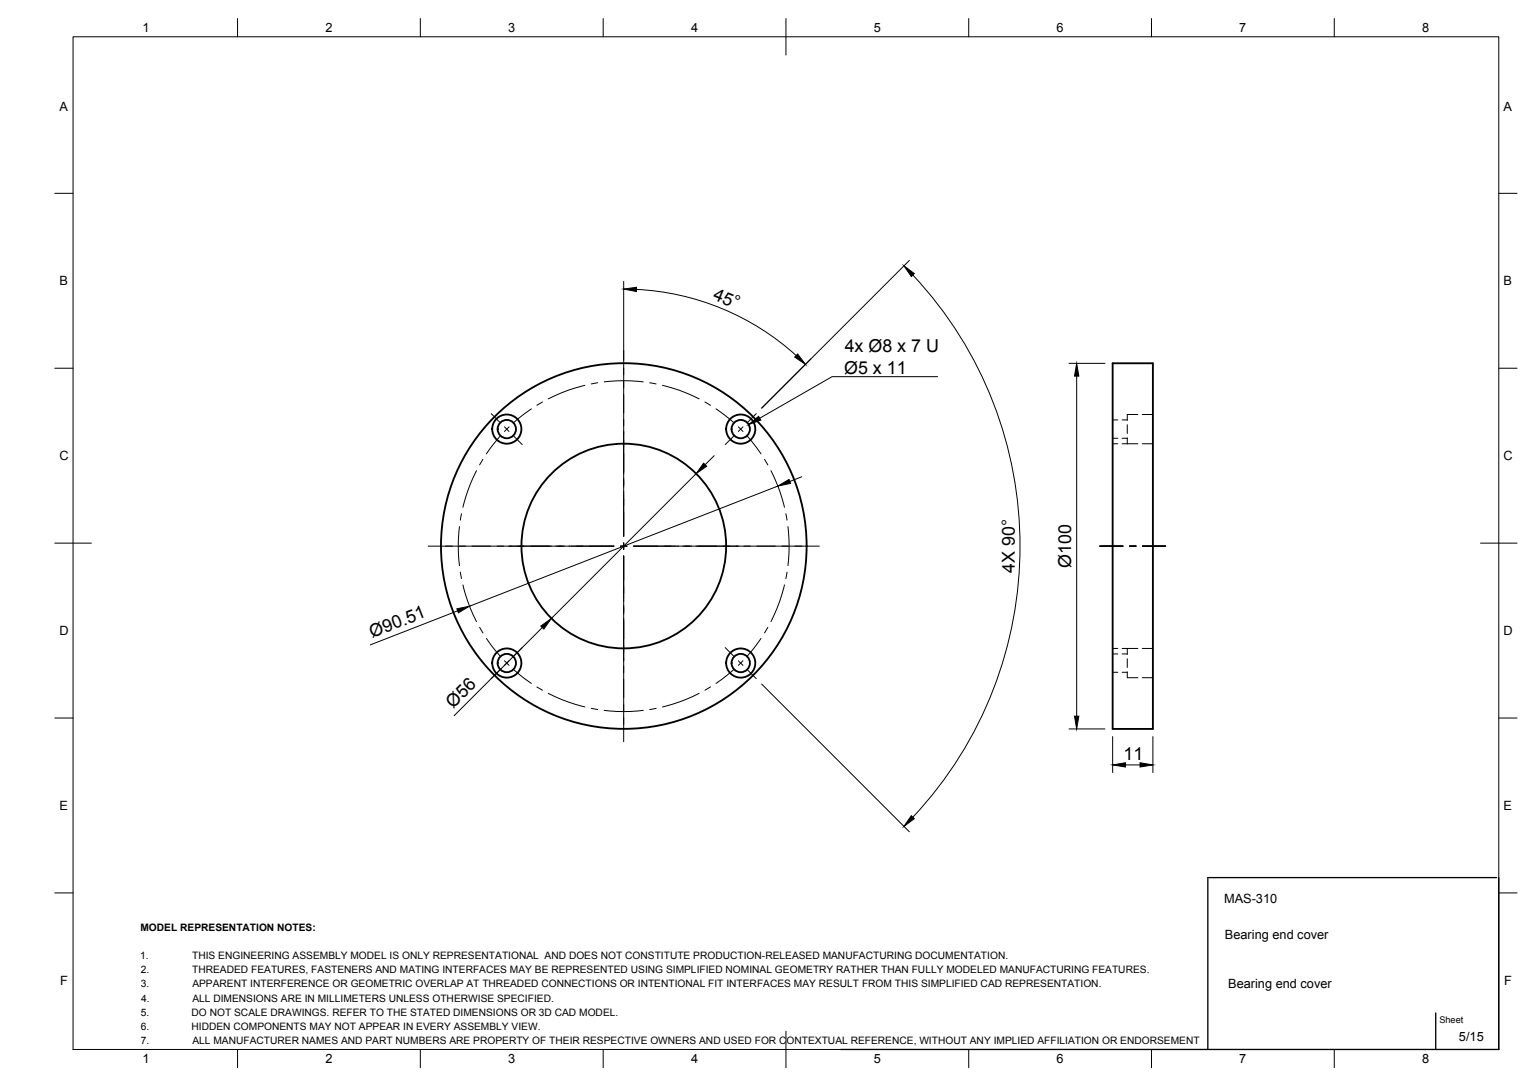
ISO-10303-21;
HEADER;
/* Generated by software containing ST-Developer
 * from STEP Tools, Inc. (www.steptools.com) 
 */

FILE_DESCRIPTION(
/* description */ ('Independent30mm screw-fed quill/spindle unit with16mm straight tool s
ocket, radial set screw, native reusable open ball bearings, retained 
inner/outer race stacks, keyed quill guide and M12x1.75 fine feed. Ext
ernal moving drive and tool not included. Ideal cage orbital links; in
dividual ball spin, force and preload not simulated. No drilling capac
ity, runout, speed, torque, load, life or machine safety rating.'),
/* implementation_level */ '2;1');

FILE_NAME(
/* name */ 'Bearing end cover.step',
/* time_stamp */ '2026-11-08T18:59:42-08:00',
/* author */ (''),
/* organization */ (''),
/* preprocessor_version */ 'ST-DEVELOPER v20.2',
/* originating_system */ 'Autodesk Translation Framework v15.17.0.0',
/* authorisation */ '');

FILE_SCHEMA (('AUTOMOTIVE_DESIGN { 1 0 10303 214 3 1 1 }'));
ENDSEC;

DATA;
#10=MECHANICAL_DESIGN_GEOMETRIC_PRESENTATION_REPRESENTATION('',(#1603),#63898);
#1567=SHAPE_REPRESENTATION_RELATIONSHIP('SRR','None',#64006,#1585);
#1585=ADVANCED_BREP_SHAPE_REPRESENTATION('',(#1621),#63891);
#1603=STYLED_ITEM('',(#64101),#1621);
#1621=MANIFOLD_SOLID_BREP('Body1',#15489);
#1692=FACE_BOUND('',#4293,.T.);
#1693=FACE_BOUND('',#4297,.T.);
#1694=FACE_BOUND('',#4301,.T.);
#1695=FACE_BOUND('',#4305,.T.);
#1696=FACE_BOUND('',#4311,.T.);
#1697=FACE_BOUND('',#4312,.T.);
#1698=FACE_BOUND('',#4313,.T.);
#1699=FACE_BOUND('',#4314,.T.);
#1700=FACE_BOUND('',#4315,.T.);
#1701=FACE_BOUND('',#4317,.T.);
#1702=FACE_BOUND('',#4318,.T.);
#1703=FACE_BOUND('',#4319,.T.);
#1704=FACE_BOUND('',#4320,.T.);
#1705=FACE_BOUND('',#4321,.T.);
#2325=CYLINDRICAL_SURFACE('',#16587,4.);
#2326=CYLINDRICAL_SURFACE('',#16589,2.5);
#2327=CYLINDRICAL_SURFACE('',#16594,4.);
#2328=CYLINDRICAL_SURFACE('',#16596,2.5);
#2329=CYLINDRICAL_SURFACE('',#16601,4.);
#2330=CYLINDRICAL_SURFACE('',#16603,2.5);
#2331=CYLINDRICAL_SURFACE('',#16608,4.);
#2332=CYLINDRICAL_SURFACE('',#16610,2.5);
#2333=CYLINDRICAL_SURFACE('',#16612,28.);
#2334=CYLINDRICAL_SURFACE('',#16615,50.);
#2550=CIRCLE('',#16585,4.);
#2551=CIRCLE('',#16586,2.5);
#2552=CIRCLE('',#16588,4.);
#2553=CIRCLE('',#16590,2.5);
#2554=CIRCLE('',#16592,4.);
#2555=CIRCLE('',#16593,2.5);
#2556=CIRCLE('',#16595,4.);
#2557=CIRCLE('',#16597,2.5);
#2558=CIRCLE('',#16599,4.);
#2559=CIRCLE('',#16600,2.5);
#2560=CIRCLE('',#16602,4.);
#2561=CIRCLE('',#16604,2.5);
#2562=CIRCLE('',#16606,4.);
#2563=CIRCLE('',#16607,2.5);
#2564=CIRCLE('',#16609,4.);
#2565=CIRCLE('',#16611,2.5);
#2566=CIRCLE('',#16613,28.);
#2567=CIRCLE('',#16614,28.);
#2568=CIRCLE('',#16616,50.);
#2569=CIRCLE('',#16617,50.);
#3390=FACE_OUTER_BOUND('',#4292,.T.);
#3391=FACE_OUTER_BOUND('',#4294,.T.);
#3392=FACE_OUTER_BOUND('',#4295,.T.);
#3393=FACE_OUTER_BOUND('',#4296,.T.);
#3394=FACE_OUTER_BOUND('',#4298,.T.);
#3395=FACE_OUTER_BOUND('',#4299,.T.);
#3396=FACE_OUTER_BOUND('',#4300,.T.);
#3397=FACE_OUTER_BOUND('',#4302,.T.);
#3398=FACE_OUTER_BOUND('',#4303,.T.);
#3399=FACE_OUTER_BOUND('',#4304,.T.);
#3400=FACE_OUTER_BOUND('',#4306,.T.);
#3401=FACE_OUTER_BOUND('',#4307,.T.);
#3402=FACE_OUTER_BOUND('',#4308,.T.);
#3403=FACE_OUTER_BOUND('',#4309,.T.);
#3404=FACE_OUTER_BOUND('',#4310,.T.);
#3405=FACE_OUTER_BOUND('',#4316,.T.);
#4292=EDGE_LOOP('',(#13930));
#4293=EDGE_LOOP('',(#13931));
#4294=EDGE_LOOP('',(#13932,#13933,#13934,#13935));
#4295=EDGE_LOOP('',(#13936,#13937,#13938,#13939));
#4296=EDGE_LOOP('',(#13940));
#4297=EDGE_LOOP('',(#13941));
#4298=EDGE_LOOP('',(#13942,#13943,#13944,#13945));
#4299=EDGE_LOOP('',(#13946,#13947,#13948,#13949));
#4300=EDGE_LOOP('',(#13950));
#4301=EDGE_LOOP('',(#13951));
#4302=EDGE_LOOP('',(#13952,#13953,#13954,#13955));
#4303=EDGE_LOOP('',(#13956,#13957,#13958,#13959));
#4304=EDGE_LOOP('',(#13960));
#4305=EDGE_LOOP('',(#13961));
#4306=EDGE_LOOP('',(#13962,#13963,#13964,#13965));
#4307=EDGE_LOOP('',(#13966,#13967,#13968,#13969));
#4308=EDGE_LOOP('',(#13970,#13971,#13972,#13973));
#4309=EDGE_LOOP('',(#13974,#13975,#13976,#13977));
#4310=EDGE_LOOP('',(#13978));
#4311=EDGE_LOOP('',(#13979));
#4312=EDGE_LOOP('',(#13980));
#4313=EDGE_LOOP('',(#13981));
#4314=EDGE_LOOP('',(#13982));
#4315=EDGE_LOOP('',(#13983));
#4316=EDGE_LOOP('',(#13984));
#4317=EDGE_LOOP('',(#13985));
#4318=EDGE_LOOP('',(#13986));
#4319=EDGE_LOOP('',(#13987));
#4320=EDGE_LOOP('',(#13988));
#4321=EDGE_LOOP('',(#13989));
#5114=LINE('',#60321,#5877);
#5115=LINE('',#60324,#5878);
#5116=LINE('',#60334,#5879);
#5117=LINE('',#60337,#5880);
#5118=LINE('',#60347,#5881);
#5119=LINE('',#60350,#5882);
#5120=LINE('',#60360,#5883);
#5121=LINE('',#60363,#5884);
#5122=LINE('',#60369,#5885);
#5123=LINE('',#60375,#5886);
#5877=VECTOR('',#19338,4.);
#5878=VECTOR('',#19341,2.5);
#5879=VECTOR('',#19354,4.);
#5880=VECTOR('',#19357,2.5);
#5881=VECTOR('',#19370,4.);
#5882=VECTOR('',#19373,2.5);
#5883=VECTOR('',#19386,4.);
#5884=VECTOR('',#19389,2.5);
#5885=VECTOR('',#19396,28.);
#5886=VECTOR('',#19403,50.);
#7310=VERTEX_POINT('',#60314);
#7311=VERTEX_POINT('',#60316);
#7312=VERTEX_POINT('',#60319);
#7313=VERTEX_POINT('',#60323);
#7314=VERTEX_POINT('',#60327);
#7315=VERTEX_POINT('',#60329);
#7316=VERTEX_POINT('',#60332);
#7317=VERTEX_POINT('',#60336);
#7318=VERTEX_POINT('',#60340);
#7319=VERTEX_POINT('',#60342);
#7320=VERTEX_POINT('',#60345);
#7321=VERTEX_POINT('',#60349);
#7322=VERTEX_POINT('',#60353);
#7323=VERTEX_POINT('',#60355);
#7324=VERTEX_POINT('',#60358);
#7325=VERTEX_POINT('',#60362);
#7326=VERTEX_POINT('',#60366);
#7327=VERTEX_POINT('',#60368);
#7328=VERTEX_POINT('',#60372);
#7329=VERTEX_POINT('',#60374);
#9554=EDGE_CURVE('',#7310,#7310,#2550,.T.);
#9555=EDGE_CURVE('',#7311,#7311,#2551,.T.);
#9556=EDGE_CURVE('',#7312,#7312,#2552,.T.);
#9557=EDGE_CURVE('',#7312,#7310,#5114,.T.);
#9558=EDGE_CURVE('',#7311,#7313,#5115,.T.);
#9559=EDGE_CURVE('',#7313,#7313,#2553,.T.);
#9560=EDGE_CURVE('',#7314,#7314,#2554,.T.);
#9561=EDGE_CURVE('',#7315,#7315,#2555,.T.);
#9562=EDGE_CURVE('',#7316,#7316,#2556,.T.);
#9563=EDGE_CURVE('',#7316,#7314,#5116,.T.);
#9564=EDGE_CURVE('',#7315,#7317,#5117,.T.);
#9565=EDGE_CURVE('',#7317,#7317,#2557,.T.);
#9566=EDGE_CURVE('',#7318,#7318,#2558,.T.);
#9567=EDGE_CURVE('',#7319,#7319,#2559,.T.);
#9568=EDGE_CURVE('',#7320,#7320,#2560,.T.);
#9569=EDGE_CURVE('',#7320,#7318,#5118,.T.);
#9570=EDGE_CURVE('',#7319,#7321,#5119,.T.);
#9571=EDGE_CURVE('',#7321,#7321,#2561,.T.);
#9572=EDGE_CURVE('',#7322,#7322,#2562,.T.);
#9573=EDGE_CURVE('',#7323,#7323,#2563,.T.);
#9574=EDGE_CURVE('',#7324,#7324,#2564,.T.);
#9575=EDGE_CURVE('',#7324,#7322,#5120,.T.);
#9576=EDGE_CURVE('',#7323,#7325,#5121,.T.);
#9577=EDGE_CURVE('',#7325,#7325,#2565,.T.);
#9578=EDGE_CURVE('',#7326,#7326,#2566,.T.);
#9579=EDGE_CURVE('',#7326,#7327,#5122,.T.);
#9580=EDGE_CURVE('',#7327,#7327,#2567,.T.);
#9581=EDGE_CURVE('',#7328,#7328,#2568,.T.);
#9582=EDGE_CURVE('',#7328,#7329,#5123,.T.);
#9583=EDGE_CURVE('',#7329,#7329,#2569,.T.);
#13930=ORIENTED_EDGE('',*,*,#9554,.F.);
#13931=ORIENTED_EDGE('',*,*,#9555,.T.);
#13932=ORIENTED_EDGE('',*,*,#9556,.F.);
#13933=ORIENTED_EDGE('',*,*,#9557,.T.);
#13934=ORIENTED_EDGE('',*,*,#9554,.T.);
#13935=ORIENTED_EDGE('',*,*,#9557,.F.);
#13936=ORIENTED_EDGE('',*,*,#9555,.F.);
#13937=ORIENTED_EDGE('',*,*,#9558,.T.);
#13938=ORIENTED_EDGE('',*,*,#9559,.F.);
#13939=ORIENTED_EDGE('',*,*,#9558,.F.);
#13940=ORIENTED_EDGE('',*,*,#9560,.F.);
#13941=ORIENTED_EDGE('',*,*,#9561,.T.);
#13942=ORIENTED_EDGE('',*,*,#9562,.F.);
#13943=ORIENTED_EDGE('',*,*,#9563,.T.);
#13944=ORIENTED_EDGE('',*,*,#9560,.T.);
#13945=ORIENTED_EDGE('',*,*,#9563,.F.);
#13946=ORIENTED_EDGE('',*,*,#9561,.F.);
#13947=ORIENTED_EDGE('',*,*,#9564,.T.);
#13948=ORIENTED_EDGE('',*,*,#9565,.F.);
#13949=ORIENTED_EDGE('',*,*,#9564,.F.);
#13950=ORIENTED_EDGE('',*,*,#9566,.F.);
#13951=ORIENTED_EDGE('',*,*,#9567,.T.);
#13952=ORIENTED_EDGE('',*,*,#9568,.F.);
#13953=ORIENTED_EDGE('',*,*,#9569,.T.);
#13954=ORIENTED_EDGE('',*,*,#9566,.T.);
#13955=ORIENTED_EDGE('',*,*,#9569,.F.);
#13956=ORIENTED_EDGE('',*,*,#9567,.F.);
#13957=ORIENTED_EDGE('',*,*,#9570,.T.);
#13958=ORIENTED_EDGE('',*,*,#9571,.F.);
#13959=ORIENTED_EDGE('',*,*,#9570,.F.);
#13960=ORIENTED_EDGE('',*,*,#9572,.F.);
#13961=ORIENTED_EDGE('',*,*,#9573,.T.);
#13962=ORIENTED_EDGE('',*,*,#9574,.F.);
#13963=ORIENTED_EDGE('',*,*,#9575,.T.);
#13964=ORIENTED_EDGE('',*,*,#9572,.T.);
#13965=ORIENTED_EDGE('',*,*,#9575,.F.);
#13966=ORIENTED_EDGE('',*,*,#9573,.F.);
#13967=ORIENTED_EDGE('',*,*,#9576,.T.);
#13968=ORIENTED_EDGE('',*,*,#9577,.F.);
#13969=ORIENTED_EDGE('',*,*,#9576,.F.);
#13970=ORIENTED_EDGE('',*,*,#9578,.F.);
#13971=ORIENTED_EDGE('',*,*,#9579,.T.);
#13972=ORIENTED_EDGE('',*,*,#9580,.T.);
#13973=ORIENTED_EDGE('',*,*,#9579,.F.);
#13974=ORIENTED_EDGE('',*,*,#9581,.F.);
#13975=ORIENTED_EDGE('',*,*,#9582,.T.);
#13976=ORIENTED_EDGE('',*,*,#9583,.T.);
#13977=ORIENTED_EDGE('',*,*,#9582,.F.);
#13978=ORIENTED_EDGE('',*,*,#9581,.T.);
#13979=ORIENTED_EDGE('',*,*,#9578,.T.);
#13980=ORIENTED_EDGE('',*,*,#9574,.T.);
#13981=ORIENTED_EDGE('',*,*,#9568,.T.);
#13982=ORIENTED_EDGE('',*,*,#9562,.T.);
#13983=ORIENTED_EDGE('',*,*,#9556,.T.);
#13984=ORIENTED_EDGE('',*,*,#9583,.F.);
#13985=ORIENTED_EDGE('',*,*,#9580,.F.);
#13986=ORIENTED_EDGE('',*,*,#9577,.T.);
#13987=ORIENTED_EDGE('',*,*,#9571,.T.);
#13988=ORIENTED_EDGE('',*,*,#9565,.T.);
#13989=ORIENTED_EDGE('',*,*,#9559,.T.);
#14605=PLANE('',#16584);
#14606=PLANE('',#16591);
#14607=PLANE('',#16598);
#14608=PLANE('',#16605);
#14609=PLANE('',#16618);
#14610=PLANE('',#16619);
#15370=ADVANCED_FACE('',(#3390,#1692),#14605,.F.);
#15371=ADVANCED_FACE('',(#3391),#2325,.F.);
#15372=ADVANCED_FACE('',(#3392),#2326,.F.);
#15373=ADVANCED_FACE('',(#3393,#1693),#14606,.F.);
#15374=ADVANCED_FACE('',(#3394),#2327,.F.);
#15375=ADVANCED_FACE('',(#3395),#2328,.F.);
#15376=ADVANCED_FACE('',(#3396,#1694),#14607,.F.);
#15377=ADVANCED_FACE('',(#3397),#2329,.F.);
#15378=ADVANCED_FACE('',(#3398),#2330,.F.);
#15379=ADVANCED_FACE('',(#3399,#1695),#14608,.F.);
#15380=ADVANCED_FACE('',(#3400),#2331,.F.);
#15381=ADVANCED_FACE('',(#3401),#2332,.F.);
#15382=ADVANCED_FACE('',(#3402),#2333,.F.);
#15383=ADVANCED_FACE('',(#3403),#2334,.T.);
#15384=ADVANCED_FACE('',(#3404,#1696,#1697,#1698,#1699,#1700),#14609,.T.);
#15385=ADVANCED_FACE('',(#3405,#1701,#1702,#1703,#1704,#1705),#14610,.F.);
#15489=CLOSED_SHELL('',(#15370,#15371,#15372,#15373,#15374,#15375,#15376,
#15377,#15378,#15379,#15380,#15381,#15382,#15383,#15384,#15385));
#16583=AXIS2_PLACEMENT_3D('',#60312,#19326,#19327);
#16584=AXIS2_PLACEMENT_3D('',#60313,#19328,#19329);
#16585=AXIS2_PLACEMENT_3D('',#60315,#19330,#19331);
#16586=AXIS2_PLACEMENT_3D('',#60317,#19332,#19333);
#16587=AXIS2_PLACEMENT_3D('',#60318,#19334,#19335);
#16588=AXIS2_PLACEMENT_3D('',#60320,#19336,#19337);
#16589=AXIS2_PLACEMENT_3D('',#60322,#19339,#19340);
#16590=AXIS2_PLACEMENT_3D('',#60325,#19342,#19343);
#16591=AXIS2_PLACEMENT_3D('',#60326,#19344,#19345);
#16592=AXIS2_PLACEMENT_3D('',#60328,#19346,#19347);
#16593=AXIS2_PLACEMENT_3D('',#60330,#19348,#19349);
#16594=AXIS2_PLACEMENT_3D('',#60331,#19350,#19351);
#16595=AXIS2_PLACEMENT_3D('',#60333,#19352,#19353);
#16596=AXIS2_PLACEMENT_3D('',#60335,#19355,#19356);
#16597=AXIS2_PLACEMENT_3D('',#60338,#19358,#19359);
#16598=AXIS2_PLACEMENT_3D('',#60339,#19360,#19361);
#16599=AXIS2_PLACEMENT_3D('',#60341,#19362,#19363);
#16600=AXIS2_PLACEMENT_3D('',#60343,#19364,#19365);
#16601=AXIS2_PLACEMENT_3D('',#60344,#19366,#19367);
#16602=AXIS2_PLACEMENT_3D('',#60346,#19368,#19369);
#16603=AXIS2_PLACEMENT_3D('',#60348,#19371,#19372);
#16604=AXIS2_PLACEMENT_3D('',#60351,#19374,#19375);
#16605=AXIS2_PLACEMENT_3D('',#60352,#19376,#19377);
#16606=AXIS2_PLACEMENT_3D('',#60354,#19378,#19379);
#16607=AXIS2_PLACEMENT_3D('',#60356,#19380,#19381);
#16608=AXIS2_PLACEMENT_3D('',#60357,#19382,#19383);
#16609=AXIS2_PLACEMENT_3D('',#60359,#19384,#19385);
#16610=AXIS2_PLACEMENT_3D('',#60361,#19387,#19388);
#16611=AXIS2_PLACEMENT_3D('',#60364,#19390,#19391);
#16612=AXIS2_PLACEMENT_3D('',#60365,#19392,#19393);
#16613=AXIS2_PLACEMENT_3D('',#60367,#19394,#19395);
#16614=AXIS2_PLACEMENT_3D('',#60370,#19397,#19398);
#16615=AXIS2_PLACEMENT_3D('',#60371,#19399,#19400);
#16616=AXIS2_PLACEMENT_3D('',#60373,#19401,#19402);
#16617=AXIS2_PLACEMENT_3D('',#60376,#19404,#19405);
#16618=AXIS2_PLACEMENT_3D('',#60377,#19406,#19407);
#16619=AXIS2_PLACEMENT_3D('',#60378,#19408,#19409);
#19326=DIRECTION('axis',(0.,0.,1.));
#19327=DIRECTION('refdir',(1.,0.,0.));
#19328=DIRECTION('center_axis',(0.,0.,-1.));
#19329=DIRECTION('ref_axis',(1.,0.,0.));
#19330=DIRECTION('center_axis',(0.,0.,-1.));
#19331=DIRECTION('ref_axis',(1.,0.,0.));
#19332=DIRECTION('center_axis',(0.,0.,-1.));
#19333=DIRECTION('ref_axis',(1.,0.,0.));
#19334=DIRECTION('center_axis',(0.,0.,-1.));
#19335=DIRECTION('ref_axis',(1.,0.,0.));
#19336=DIRECTION('center_axis',(0.,0.,-1.));
#19337=DIRECTION('ref_axis',(1.,0.,0.));
#19338=DIRECTION('',(0.,0.,-1.));
#19339=DIRECTION('center_axis',(0.,0.,-1.));
#19340=DIRECTION('ref_axis',(1.,0.,0.));
#19341=DIRECTION('',(0.,0.,-1.));
#19342=DIRECTION('center_axis',(0.,0.,1.));
#19343=DIRECTION('ref_axis',(1.,0.,0.));
#19344=DIRECTION('center_axis',(0.,0.,-1.));
#19345=DIRECTION('ref_axis',(1.,0.,0.));
#19346=DIRECTION('center_axis',(0.,0.,-1.));
#19347=DIRECTION('ref_axis',(1.,0.,0.));
#19348=DIRECTION('center_axis',(0.,0.,-1.));
#19349=DIRECTION('ref_axis',(1.,0.,0.));
#19350=DIRECTION('center_axis',(0.,0.,-1.));
#19351=DIRECTION('ref_axis',(1.,0.,0.));
#19352=DIRECTION('center_axis',(0.,0.,-1.));
#19353=DIRECTION('ref_axis',(1.,0.,0.));
#19354=DIRECTION('',(0.,0.,-1.));
#19355=DIRECTION('center_axis',(0.,0.,-1.));
#19356=DIRECTION('ref_axis',(1.,0.,0.));
#19357=DIRECTION('',(0.,0.,-1.));
#19358=DIRECTION('center_axis',(0.,0.,1.));
#19359=DIRECTION('ref_axis',(1.,0.,0.));
#19360=DIRECTION('center_axis',(0.,0.,-1.));
#19361=DIRECTION('ref_axis',(1.,0.,0.));
#19362=DIRECTION('center_axis',(0.,0.,-1.));
#19363=DIRECTION('ref_axis',(1.,0.,0.));
#19364=DIRECTION('center_axis',(0.,0.,-1.));
#19365=DIRECTION('ref_axis',(1.,0.,0.));
#19366=DIRECTION('center_axis',(0.,0.,-1.));
#19367=DIRECTION('ref_axis',(1.,0.,0.));
#19368=DIRECTION('center_axis',(0.,0.,-1.));
#19369=DIRECTION('ref_axis',(1.,0.,0.));
#19370=DIRECTION('',(0.,0.,-1.));
#19371=DIRECTION('center_axis',(0.,0.,-1.));
#19372=DIRECTION('ref_axis',(1.,0.,0.));
#19373=DIRECTION('',(0.,0.,-1.));
#19374=DIRECTION('center_axis',(0.,0.,1.));
#19375=DIRECTION('ref_axis',(1.,0.,0.));
#19376=DIRECTION('center_axis',(0.,0.,-1.));
#19377=DIRECTION('ref_axis',(1.,0.,0.));
#19378=DIRECTION('center_axis',(0.,0.,-1.));
#19379=DIRECTION('ref_axis',(1.,0.,0.));
#19380=DIRECTION('center_axis',(0.,0.,-1.));
#19381=DIRECTION('ref_axis',(1.,0.,0.));
#19382=DIRECTION('center_axis',(0.,0.,-1.));
#19383=DIRECTION('ref_axis',(1.,0.,0.));
#19384=DIRECTION('center_axis',(0.,0.,-1.));
#19385=DIRECTION('ref_axis',(1.,0.,0.));
#19386=DIRECTION('',(0.,0.,-1.));
#19387=DIRECTION('center_axis',(0.,0.,-1.));
#19388=DIRECTION('ref_axis',(1.,0.,0.));
#19389=DIRECTION('',(0.,0.,-1.));
#19390=DIRECTION('center_axis',(0.,0.,1.));
#19391=DIRECTION('ref_axis',(1.,0.,0.));
#19392=DIRECTION('center_axis',(0.,0.,1.));
#19393=DIRECTION('ref_axis',(1.,0.,0.));
#19394=DIRECTION('center_axis',(0.,0.,-1.));
#19395=DIRECTION('ref_axis',(1.,0.,0.));
#19396=DIRECTION('',(0.,0.,-1.));
#19397=DIRECTION('center_axis',(0.,0.,-1.));
#19398=DIRECTION('ref_axis',(1.,0.,0.));
#19399=DIRECTION('center_axis',(0.,0.,1.));
#19400=DIRECTION('ref_axis',(1.,0.,0.));
#19401=DIRECTION('center_axis',(0.,0.,1.));
#19402=DIRECTION('ref_axis',(1.,0.,0.));
#19403=DIRECTION('',(0.,0.,-1.));
#19404=DIRECTION('center_axis',(0.,0.,1.));
#19405=DIRECTION('ref_axis',(1.,0.,0.));
#19406=DIRECTION('center_axis',(0.,0.,1.));
#19407=DIRECTION('ref_axis',(1.,0.,0.));
#19408=DIRECTION('center_axis',(0.,0.,1.));
#19409=DIRECTION('ref_axis',(1.,0.,0.));
#60312=CARTESIAN_POINT('',(0.,0.,0.));
#60313=CARTESIAN_POINT('Origin',(32.,-32.,4.));
#60314=CARTESIAN_POINT('',(28.,-32.,4.));
#60315=CARTESIAN_POINT('Origin',(32.,-32.,4.));
#60316=CARTESIAN_POINT('',(29.5,-32.,4.));
#60317=CARTESIAN_POINT('Origin',(32.,-32.,4.));
#60318=CARTESIAN_POINT('Origin',(32.,-32.,7.5));
#60319=CARTESIAN_POINT('',(28.,-32.,11.));
#60320=CARTESIAN_POINT('Origin',(32.,-32.,11.));
#60321=CARTESIAN_POINT('',(28.,-32.,7.5));
#60322=CARTESIAN_POINT('Origin',(32.,-32.,5.5));
#60323=CARTESIAN_POINT('',(29.5,-32.,0.));
#60324=CARTESIAN_POINT('',(29.5,-32.,5.5));
#60325=CARTESIAN_POINT('Origin',(32.,-32.,0.));
#60326=CARTESIAN_POINT('Origin',(-32.,-32.,4.));
#60327=CARTESIAN_POINT('',(-36.,-32.,4.));
#60328=CARTESIAN_POINT('Origin',(-32.,-32.,4.));
#60329=CARTESIAN_POINT('',(-34.5,-32.,4.));
#60330=CARTESIAN_POINT('Origin',(-32.,-32.,4.));
#60331=CARTESIAN_POINT('Origin',(-32.,-32.,7.5));
#60332=CARTESIAN_POINT('',(-36.,-32.,11.));
#60333=CARTESIAN_POINT('Origin',(-32.,-32.,11.));
#60334=CARTESIAN_POINT('',(-36.,-32.,7.5));
#60335=CARTESIAN_POINT('Origin',(-32.,-32.,5.5));
#60336=CARTESIAN_POINT('',(-34.5,-32.,0.));
#60337=CARTESIAN_POINT('',(-34.5,-32.,5.5));
#60338=CARTESIAN_POINT('Origin',(-32.,-32.,0.));
#60339=CARTESIAN_POINT('Origin',(-32.,32.,4.));
#60340=CARTESIAN_POINT('',(-36.,32.,4.));
#60341=CARTESIAN_POINT('Origin',(-32.,32.,4.));
#60342=CARTESIAN_POINT('',(-34.5,32.,4.));
#60343=CARTESIAN_POINT('Origin',(-32.,32.,4.));
#60344=CARTESIAN_POINT('Origin',(-32.,32.,7.5));
#60345=CARTESIAN_POINT('',(-36.,32.,11.));
#60346=CARTESIAN_POINT('Origin',(-32.,32.,11.));
#60347=CARTESIAN_POINT('',(-36.,32.,7.5));
#60348=CARTESIAN_POINT('Origin',(-32.,32.,5.5));
#60349=CARTESIAN_POINT('',(-34.5,32.,0.));
#60350=CARTESIAN_POINT('',(-34.5,32.,5.5));
#60351=CARTESIAN_POINT('Origin',(-32.,32.,0.));
#60352=CARTESIAN_POINT('Origin',(32.,32.,4.));
#60353=CARTESIAN_POINT('',(28.,32.,4.));
#60354=CARTESIAN_POINT('Origin',(32.,32.,4.));
#60355=CARTESIAN_POINT('',(29.5,32.,4.));
#60356=CARTESIAN_POINT('Origin',(32.,32.,4.));
#60357=CARTESIAN_POINT('Origin',(32.,32.,7.5));
#60358=CARTESIAN_POINT('',(28.,32.,11.));
#60359=CARTESIAN_POINT('Origin',(32.,32.,11.));
#60360=CARTESIAN_POINT('',(28.,32.,7.5));
#60361=CARTESIAN_POINT('Origin',(32.,32.,5.5));
#60362=CARTESIAN_POINT('',(29.5,32.,0.));
#60363=CARTESIAN_POINT('',(29.5,32.,5.5));
#60364=CARTESIAN_POINT('Origin',(32.,32.,0.));
#60365=CARTESIAN_POINT('Origin',(0.,0.,0.));
#60366=CARTESIAN_POINT('',(-28.,-3.42901103761259E-15,11.));
#60367=CARTESIAN_POINT('Origin',(0.,0.,11.));
#60368=CARTESIAN_POINT('',(-28.,-3.42901103761259E-15,0.));
#60369=CARTESIAN_POINT('',(-28.,-3.42901103761259E-15,0.));
#60370=CARTESIAN_POINT('Origin',(0.,0.,0.));
#60371=CARTESIAN_POINT('Origin',(0.,0.,0.));
#60372=CARTESIAN_POINT('',(-50.,-6.12323399573677E-15,11.));
#60373=CARTESIAN_POINT('Origin',(0.,0.,11.));
#60374=CARTESIAN_POINT('',(-50.,-6.12323399573677E-15,0.));
#60375=CARTESIAN_POINT('',(-50.,-6.12323399573677E-15,0.));
#60376=CARTESIAN_POINT('Origin',(0.,0.,0.));
#60377=CARTESIAN_POINT('Origin',(0.,0.,11.));
#60378=CARTESIAN_POINT('Origin',(0.,0.,0.));
#63871=UNCERTAINTY_MEASURE_WITH_UNIT(LENGTH_MEASURE(0.01),#63899,
'DISTANCE_ACCURACY_VALUE',
'Maximum model space distance between geometric entities at asserted c
onnectivities');
#63878=UNCERTAINTY_MEASURE_WITH_UNIT(LENGTH_MEASURE(0.01),#63899,
'DISTANCE_ACCURACY_VALUE',
'Maximum model space distance between geometric entities at asserted c
onnectivities');
#63891=(
GEOMETRIC_REPRESENTATION_CONTEXT(3)
GLOBAL_UNCERTAINTY_ASSIGNED_CONTEXT((#63871))
GLOBAL_UNIT_ASSIGNED_CONTEXT((#63899,#63901,#63902))
REPRESENTATION_CONTEXT('','3D')
);
#63898=(
GEOMETRIC_REPRESENTATION_CONTEXT(3)
GLOBAL_UNCERTAINTY_ASSIGNED_CONTEXT((#63878))
GLOBAL_UNIT_ASSIGNED_CONTEXT((#63899,#63901,#63902))
REPRESENTATION_CONTEXT('','3D')
);
#63899=(
LENGTH_UNIT()
NAMED_UNIT(*)
SI_UNIT(.MILLI.,.METRE.)
);
#63901=(
NAMED_UNIT(*)
PLANE_ANGLE_UNIT()
SI_UNIT($,.RADIAN.)
);
#63902=(
NAMED_UNIT(*)
SI_UNIT($,.STERADIAN.)
SOLID_ANGLE_UNIT()
);
#63915=SHAPE_DEFINITION_REPRESENTATION(#63934,#64006);
#63934=PRODUCT_DEFINITION_SHAPE('',$,#64026);
#64006=SHAPE_REPRESENTATION('',(#16583),#63891);
#64013=PRODUCT_DEFINITION_CONTEXT('part definition',#64072,'design');
#64026=PRODUCT_DEFINITION('Bearing end cover','Bearing end cover',#64045,
#64013);
#64045=PRODUCT_DEFINITION_FORMATION('',$,#64086);
#64072=APPLICATION_CONTEXT(
'Core Data for Automotive Mechanical Design Process');
#64073=PRODUCT_CONTEXT('part definition',#64072,'mechanical');
#64086=PRODUCT('Bearing end cover','Bearing end cover',$,(#64073));
#64101=PRESENTATION_STYLE_ASSIGNMENT((#64114));
#64114=SURFACE_STYLE_USAGE(.BOTH.,#64127);
#64127=SURFACE_SIDE_STYLE('',(#64140));
#64140=SURFACE_STYLE_FILL_AREA(#64153);
#64153=FILL_AREA_STYLE('Sky blue',(#64166));
#64166=FILL_AREA_STYLE_COLOUR('Sky blue',#64179);
#64179=COLOUR_RGB('Sky blue',0.317647058823529,0.686274509803922,0.890196078431372);
ENDSEC;
END-ISO-10303-21;
